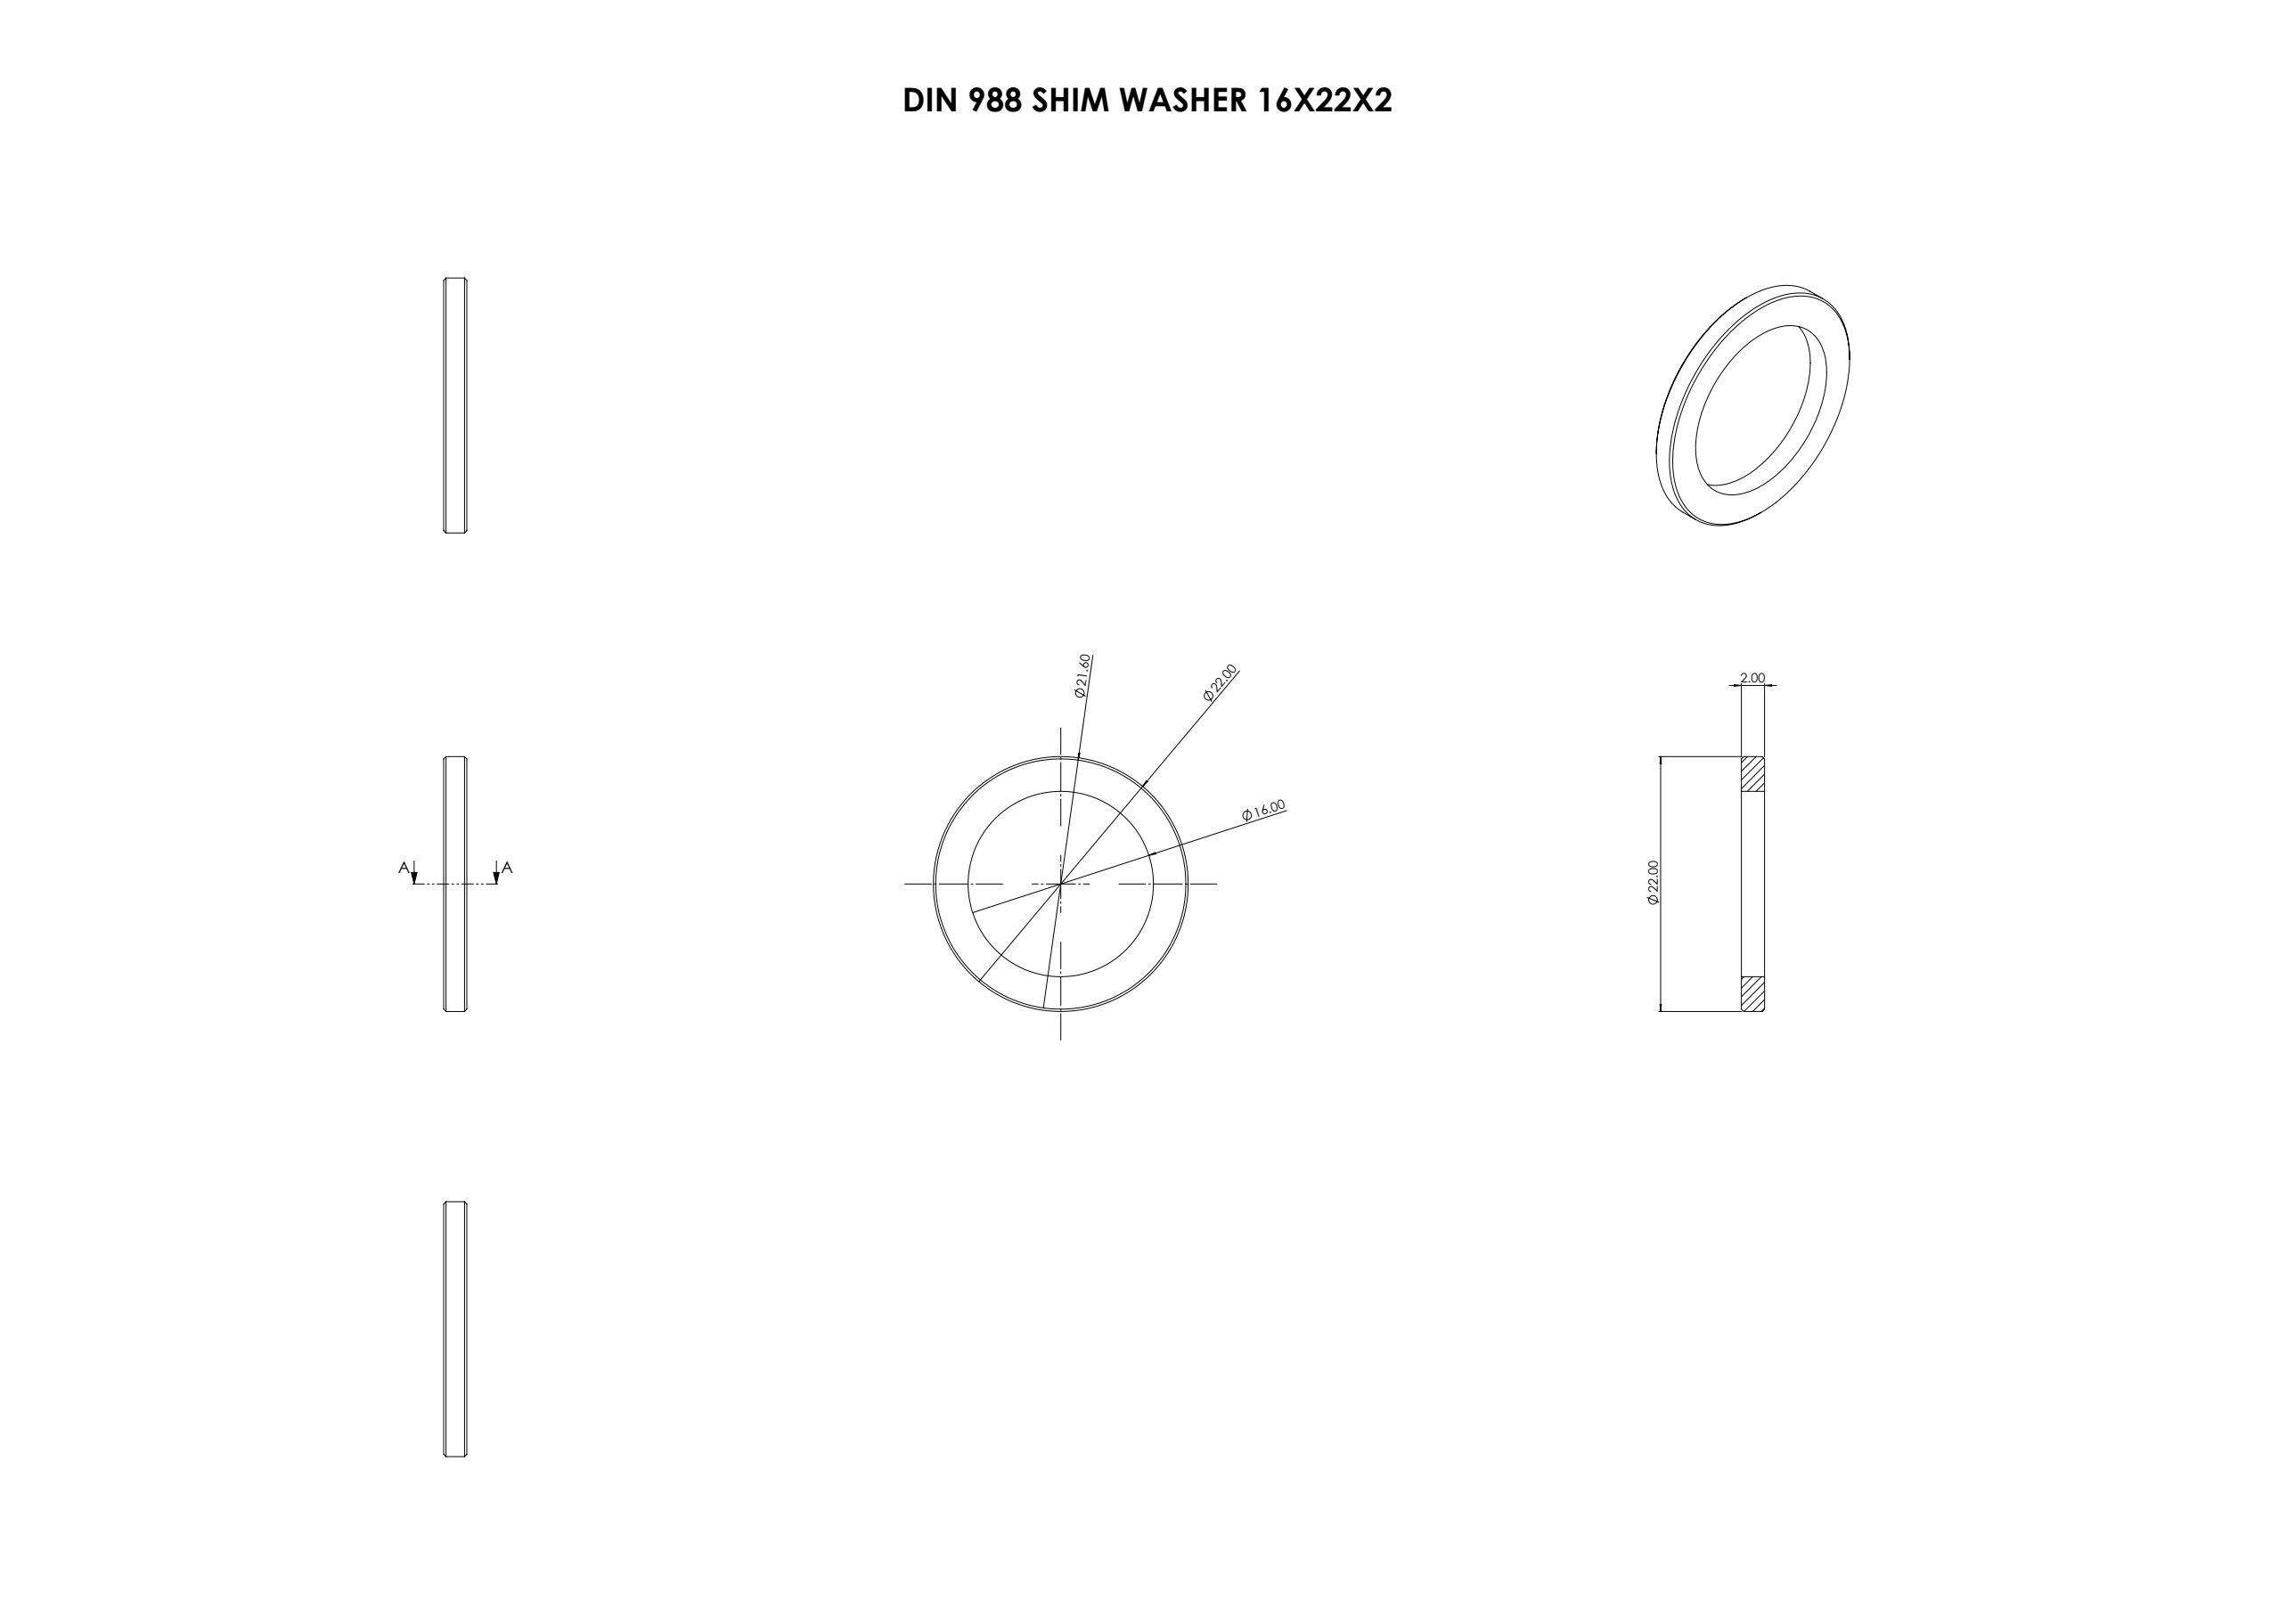
ISO-10303-21;
HEADER;
/* Generated by software containing ST-Developer
 * from STEP Tools, Inc. (www.steptools.com) 
 */

FILE_DESCRIPTION(
/* description */ (''),
/* implementation_level */ '2;1');

FILE_NAME(
/* name */ '08_DIN_988_Shim_Washer_16x22x2.step',
/* time_stamp */ '2026-10-24T13:41:11-07:00',
/* author */ (''),
/* organization */ (''),
/* preprocessor_version */ 'ST-DEVELOPER v20.2',
/* originating_system */ 'Autodesk Translation Framework v15.15.0.0',
/* authorisation */ '');

FILE_SCHEMA (('AUTOMOTIVE_DESIGN { 1 0 10303 214 3 1 1 }'));
ENDSEC;

DATA;
#10=MECHANICAL_DESIGN_GEOMETRIC_PRESENTATION_REPRESENTATION('',(#128),#12813);
#99=CONICAL_SURFACE('',#4931,10.9,0.785398163397449);
#100=CONICAL_SURFACE('',#4936,10.9,0.785398163397448);
#108=SHAPE_REPRESENTATION_RELATIONSHIP('SRR','None',#12861,#118);
#118=ADVANCED_BREP_SHAPE_REPRESENTATION('',(#138),#12810);
#128=STYLED_ITEM('',(#12981),#138);
#138=MANIFOLD_SOLID_BREP('Body1',#4391);
#163=FACE_BOUND('',#846,.T.);
#164=FACE_BOUND('',#849,.T.);
#222=PLANE('',#4938);
#223=PLANE('',#4942);
#550=FACE_OUTER_BOUND('',#842,.T.);
#551=FACE_OUTER_BOUND('',#843,.T.);
#552=FACE_OUTER_BOUND('',#844,.T.);
#553=FACE_OUTER_BOUND('',#845,.T.);
#554=FACE_OUTER_BOUND('',#847,.T.);
#555=FACE_OUTER_BOUND('',#848,.T.);
#842=EDGE_LOOP('',(#3853,#3854,#3855,#3856));
#843=EDGE_LOOP('',(#3857,#3858,#3859,#3860));
#844=EDGE_LOOP('',(#3861,#3862,#3863,#3864));
#845=EDGE_LOOP('',(#3865));
#846=EDGE_LOOP('',(#3866));
#847=EDGE_LOOP('',(#3867,#3868,#3869,#3870));
#848=EDGE_LOOP('',(#3871));
#849=EDGE_LOOP('',(#3872));
#1109=CIRCLE('',#4932,11.);
#1110=CIRCLE('',#4933,10.8);
#1111=CIRCLE('',#4935,11.);
#1112=CIRCLE('',#4937,10.8);
#1113=CIRCLE('',#4939,8.);
#1114=CIRCLE('',#4941,8.);
#1279=LINE('',#12597,#1509);
#1280=LINE('',#12602,#1510);
#1281=LINE('',#12606,#1511);
#1282=LINE('',#12612,#1512);
#1509=VECTOR('',#6016,10.9);
#1510=VECTOR('',#6023,11.);
#1511=VECTOR('',#6028,10.9);
#1512=VECTOR('',#6035,8.);
#2086=VERTEX_POINT('',#12594);
#2087=VERTEX_POINT('',#12596);
#2088=VERTEX_POINT('',#12600);
#2089=VERTEX_POINT('',#12604);
#2090=VERTEX_POINT('',#12608);
#2091=VERTEX_POINT('',#12611);
#2679=EDGE_CURVE('',#2086,#2086,#1109,.T.);
#2680=EDGE_CURVE('',#2086,#2087,#1279,.T.);
#2681=EDGE_CURVE('',#2087,#2087,#1110,.T.);
#2682=EDGE_CURVE('',#2088,#2088,#1111,.T.);
#2683=EDGE_CURVE('',#2088,#2086,#1280,.T.);
#2684=EDGE_CURVE('',#2089,#2089,#1112,.T.);
#2685=EDGE_CURVE('',#2089,#2088,#1281,.T.);
#2686=EDGE_CURVE('',#2090,#2090,#1113,.T.);
#2687=EDGE_CURVE('',#2090,#2091,#1282,.T.);
#2688=EDGE_CURVE('',#2091,#2091,#1114,.T.);
#3853=ORIENTED_EDGE('',*,*,#2679,.F.);
#3854=ORIENTED_EDGE('',*,*,#2680,.T.);
#3855=ORIENTED_EDGE('',*,*,#2681,.T.);
#3856=ORIENTED_EDGE('',*,*,#2680,.F.);
#3857=ORIENTED_EDGE('',*,*,#2682,.F.);
#3858=ORIENTED_EDGE('',*,*,#2683,.T.);
#3859=ORIENTED_EDGE('',*,*,#2679,.T.);
#3860=ORIENTED_EDGE('',*,*,#2683,.F.);
#3861=ORIENTED_EDGE('',*,*,#2684,.F.);
#3862=ORIENTED_EDGE('',*,*,#2685,.T.);
#3863=ORIENTED_EDGE('',*,*,#2682,.T.);
#3864=ORIENTED_EDGE('',*,*,#2685,.F.);
#3865=ORIENTED_EDGE('',*,*,#2684,.T.);
#3866=ORIENTED_EDGE('',*,*,#2686,.F.);
#3867=ORIENTED_EDGE('',*,*,#2686,.T.);
#3868=ORIENTED_EDGE('',*,*,#2687,.T.);
#3869=ORIENTED_EDGE('',*,*,#2688,.F.);
#3870=ORIENTED_EDGE('',*,*,#2687,.F.);
#3871=ORIENTED_EDGE('',*,*,#2681,.F.);
#3872=ORIENTED_EDGE('',*,*,#2688,.T.);
#4108=CYLINDRICAL_SURFACE('',#4934,11.);
#4109=CYLINDRICAL_SURFACE('',#4940,8.);
#4340=ADVANCED_FACE('',(#550),#99,.T.);
#4341=ADVANCED_FACE('',(#551),#4108,.T.);
#4342=ADVANCED_FACE('',(#552),#100,.T.);
#4343=ADVANCED_FACE('',(#553,#163),#222,.T.);
#4344=ADVANCED_FACE('',(#554),#4109,.F.);
#4345=ADVANCED_FACE('',(#555,#164),#223,.T.);
#4391=CLOSED_SHELL('',(#4340,#4341,#4342,#4343,#4344,#4345));
#4930=AXIS2_PLACEMENT_3D('',#12592,#6010,#6011);
#4931=AXIS2_PLACEMENT_3D('',#12593,#6012,#6013);
#4932=AXIS2_PLACEMENT_3D('',#12595,#6014,#6015);
#4933=AXIS2_PLACEMENT_3D('',#12598,#6017,#6018);
#4934=AXIS2_PLACEMENT_3D('',#12599,#6019,#6020);
#4935=AXIS2_PLACEMENT_3D('',#12601,#6021,#6022);
#4936=AXIS2_PLACEMENT_3D('',#12603,#6024,#6025);
#4937=AXIS2_PLACEMENT_3D('',#12605,#6026,#6027);
#4938=AXIS2_PLACEMENT_3D('',#12607,#6029,#6030);
#4939=AXIS2_PLACEMENT_3D('',#12609,#6031,#6032);
#4940=AXIS2_PLACEMENT_3D('',#12610,#6033,#6034);
#4941=AXIS2_PLACEMENT_3D('',#12613,#6036,#6037);
#4942=AXIS2_PLACEMENT_3D('',#12614,#6038,#6039);
#6010=DIRECTION('axis',(0.,0.,1.));
#6011=DIRECTION('refdir',(1.,0.,0.));
#6012=DIRECTION('center_axis',(1.,0.,0.));
#6013=DIRECTION('ref_axis',(0.,1.,0.));
#6014=DIRECTION('center_axis',(1.,0.,0.));
#6015=DIRECTION('ref_axis',(0.,0.,-1.));
#6016=DIRECTION('',(-0.707106781186547,0.707106781186548,8.65956056235494E-17));
#6017=DIRECTION('center_axis',(1.,0.,0.));
#6018=DIRECTION('ref_axis',(0.,0.,-1.));
#6019=DIRECTION('center_axis',(1.,0.,0.));
#6020=DIRECTION('ref_axis',(0.,1.,0.));
#6021=DIRECTION('center_axis',(1.,0.,0.));
#6022=DIRECTION('ref_axis',(0.,0.,-1.));
#6023=DIRECTION('',(-1.,0.,0.));
#6024=DIRECTION('center_axis',(-1.,0.,0.));
#6025=DIRECTION('ref_axis',(0.,1.,0.));
#6026=DIRECTION('center_axis',(1.,0.,0.));
#6027=DIRECTION('ref_axis',(0.,0.,-1.));
#6028=DIRECTION('',(-0.707106781186547,-0.707106781186547,-8.65956056235493E-17));
#6029=DIRECTION('center_axis',(1.,0.,0.));
#6030=DIRECTION('ref_axis',(0.,0.,-1.));
#6031=DIRECTION('center_axis',(1.,0.,0.));
#6032=DIRECTION('ref_axis',(0.,0.,-1.));
#6033=DIRECTION('center_axis',(1.,0.,0.));
#6034=DIRECTION('ref_axis',(0.,1.,0.));
#6035=DIRECTION('',(-1.,0.,0.));
#6036=DIRECTION('center_axis',(1.,0.,0.));
#6037=DIRECTION('ref_axis',(0.,0.,-1.));
#6038=DIRECTION('center_axis',(-1.,0.,0.));
#6039=DIRECTION('ref_axis',(0.,0.,1.));
#12592=CARTESIAN_POINT('',(0.,0.,0.));
#12593=CARTESIAN_POINT('Origin',(0.1,0.,0.));
#12594=CARTESIAN_POINT('',(0.2,-11.,-1.34711147906209E-15));
#12595=CARTESIAN_POINT('Origin',(0.2,0.,0.));
#12596=CARTESIAN_POINT('',(-2.08166817117217E-16,-10.8,-1.32261854307914E-15));
#12597=CARTESIAN_POINT('',(0.1,-10.9,-1.33486501107062E-15));
#12598=CARTESIAN_POINT('Origin',(0.,0.,0.));
#12599=CARTESIAN_POINT('Origin',(1.,0.,0.));
#12600=CARTESIAN_POINT('',(1.8,-11.,-1.34711147906209E-15));
#12601=CARTESIAN_POINT('Origin',(1.8,0.,0.));
#12602=CARTESIAN_POINT('',(1.,-11.,-1.34711147906209E-15));
#12603=CARTESIAN_POINT('Origin',(1.9,0.,0.));
#12604=CARTESIAN_POINT('',(2.,-10.8,-1.32261854307914E-15));
#12605=CARTESIAN_POINT('Origin',(2.,0.,0.));
#12606=CARTESIAN_POINT('',(1.9,-10.9,-1.33486501107062E-15));
#12607=CARTESIAN_POINT('Origin',(2.,8.,0.));
#12608=CARTESIAN_POINT('',(2.,-8.,-9.79717439317883E-16));
#12609=CARTESIAN_POINT('Origin',(2.,0.,0.));
#12610=CARTESIAN_POINT('Origin',(1.,0.,0.));
#12611=CARTESIAN_POINT('',(0.,-8.,-9.79717439317883E-16));
#12612=CARTESIAN_POINT('',(1.,-8.,-9.79717439317883E-16));
#12613=CARTESIAN_POINT('Origin',(0.,0.,0.));
#12614=CARTESIAN_POINT('Origin',(0.,10.8,0.));
#12798=UNCERTAINTY_MEASURE_WITH_UNIT(LENGTH_MEASURE(0.01),#12814,
'DISTANCE_ACCURACY_VALUE',
'Maximum model space distance between geometric entities at asserted c
onnectivities');
#12801=UNCERTAINTY_MEASURE_WITH_UNIT(LENGTH_MEASURE(0.01),#12814,
'DISTANCE_ACCURACY_VALUE',
'Maximum model space distance between geometric entities at asserted c
onnectivities');
#12810=(
GEOMETRIC_REPRESENTATION_CONTEXT(3)
GLOBAL_UNCERTAINTY_ASSIGNED_CONTEXT((#12798))
GLOBAL_UNIT_ASSIGNED_CONTEXT((#12814,#12816,#12817))
REPRESENTATION_CONTEXT('','3D')
);
#12813=(
GEOMETRIC_REPRESENTATION_CONTEXT(3)
GLOBAL_UNCERTAINTY_ASSIGNED_CONTEXT((#12801))
GLOBAL_UNIT_ASSIGNED_CONTEXT((#12814,#12816,#12817))
REPRESENTATION_CONTEXT('','3D')
);
#12814=(
LENGTH_UNIT()
NAMED_UNIT(*)
SI_UNIT(.MILLI.,.METRE.)
);
#12816=(
NAMED_UNIT(*)
PLANE_ANGLE_UNIT()
SI_UNIT($,.RADIAN.)
);
#12817=(
NAMED_UNIT(*)
SI_UNIT($,.STERADIAN.)
SOLID_ANGLE_UNIT()
);
#12826=SHAPE_DEFINITION_REPRESENTATION(#12837,#12861);
#12837=PRODUCT_DEFINITION_SHAPE('',$,#12873);
#12861=SHAPE_REPRESENTATION('',(#4930),#12810);
#12864=PRODUCT_DEFINITION_CONTEXT('part definition',#12899,'design');
#12873=PRODUCT_DEFINITION('2026-10-11-12-17-36-331',
'08_DIN_988_Shim_Washer_16x22x2',#12884,#12864);
#12884=PRODUCT_DEFINITION_FORMATION('',$,#12909);
#12899=APPLICATION_CONTEXT(
'Core Data for Automotive Mechanical Design Process');
#12900=PRODUCT_CONTEXT('part definition',#12899,'mechanical');
#12909=PRODUCT('2026-10-11-12-17-36-331',
'08_DIN_988_Shim_Washer_16x22x2',$,(#12900));
#12975=COLOUR_RGB('Black',0.12,0.14,0.17);
#12976=FILL_AREA_STYLE_COLOUR('',#12975);
#12977=FILL_AREA_STYLE('',(#12976));
#12978=SURFACE_STYLE_FILL_AREA(#12977);
#12979=SURFACE_SIDE_STYLE('',(#12978));
#12980=SURFACE_STYLE_USAGE(.BOTH.,#12979);
#12981=PRESENTATION_STYLE_ASSIGNMENT((#12980));
ENDSEC;
END-ISO-10303-21;
